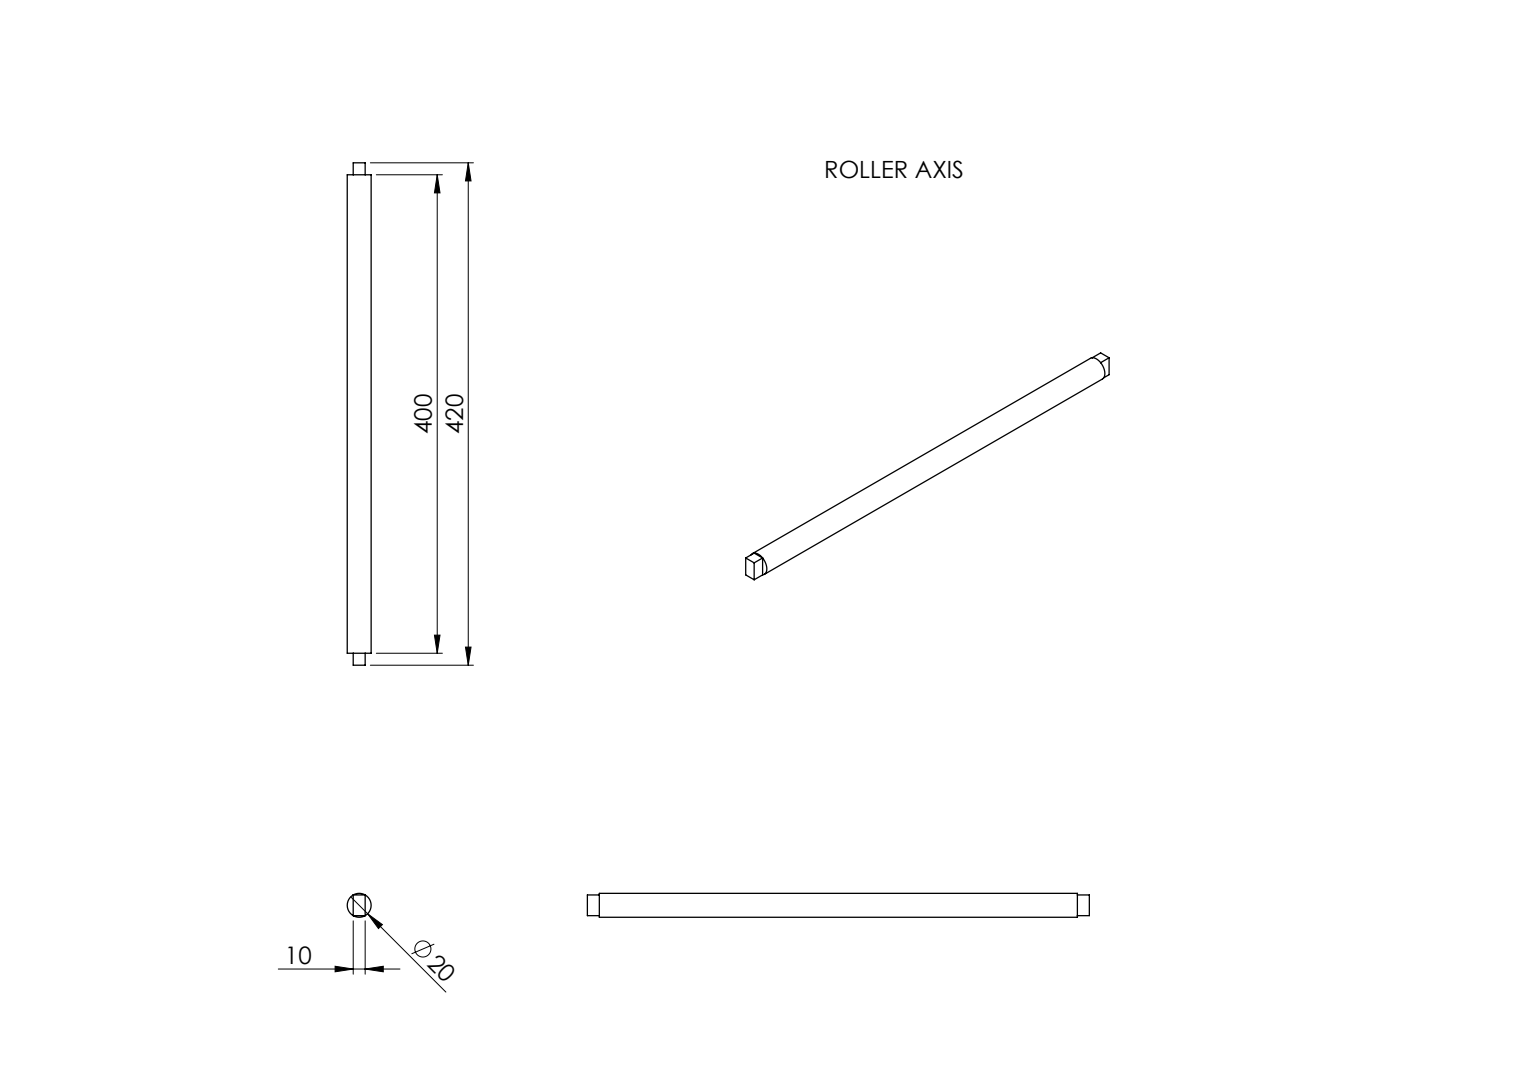
ISO-10303-21;
HEADER;
FILE_DESCRIPTION (('STEP AP214'),
    '1' );
FILE_NAME ('roller axis.step',
    '2026-10-24T13:33:06',
    ( '' ),
    ( '' ),
    'SwSTEP 2.0',
    'SolidWorks 2026',
    '' );
FILE_SCHEMA (( 'AUTOMOTIVE_DESIGN' ));
ENDSEC;

DATA;
#26=COLOUR_RGB ( '',0.8941176470588234615, 0.8941176470588234615, 0.8941176470588234615 ) ;
#48=PLANE ( 'NONE',  #10641 ) ;
#72=( NAMED_UNIT ( * ) SI_UNIT ( $, .STERADIAN. ) SOLID_ANGLE_UNIT ( ) );
#74=EDGE_CURVE ( 'NONE', #2665, #8392, #9526, .T. ) ;
#100=VECTOR ( 'NONE', #4876, 1000.000000000000000 ) ;
#101=ORIENTED_EDGE ( 'NONE', *, *, #7387, .T. ) ;
#140=VERTEX_POINT ( 'NONE', #5318 ) ;
#149=AXIS2_PLACEMENT_3D ( 'NONE', #12993, #2990, #1889 ) ;
#346=AXIS2_PLACEMENT_3D ( 'NONE', #5589, #5997, #454 ) ;
#386=VECTOR ( 'NONE', #10609, 1000.000000000000000 ) ;
#408=ORIENTED_EDGE ( 'NONE', *, *, #12527, .T. ) ;
#454=DIRECTION ( 'NONE',  ( 1.000000000000000000, 0.000000000000000000, 0.000000000000000000 ) ) ;
#467=CARTESIAN_POINT ( 'NONE',  ( 4.999999999999999112, 8.660254037844390851, 210.0000000000000000 ) ) ;
#483=PLANE ( 'NONE',  #11041 ) ;
#485=VECTOR ( 'NONE', #5913, 1000.000000000000000 ) ;
#488=CARTESIAN_POINT ( 'NONE',  ( 4.999999999999997335, -8.660254037844389075, -200.0000000000000000 ) ) ;
#527=LINE ( 'NONE', #11178, #7784 ) ;
#538=SURFACE_STYLE_FILL_AREA ( #13829 ) ;
#570=ORIENTED_EDGE ( 'NONE', *, *, #8444, .F. ) ;
#585=ORIENTED_EDGE ( 'NONE', *, *, #10780, .T. ) ;
#586=VECTOR ( 'NONE', #11904, 1000.000000000000000 ) ;
#593=AXIS2_PLACEMENT_3D ( 'NONE', #467, #9356, #3452 ) ;
#615=( NAMED_UNIT ( * ) PLANE_ANGLE_UNIT ( ) SI_UNIT ( $, .RADIAN. ) );
#620=AXIS2_PLACEMENT_3D ( 'NONE', #2454, #1137, #8922 ) ;
#723=CIRCLE ( 'NONE', #11163, 10.00000000000000000 ) ;
#735=AXIS2_PLACEMENT_3D ( 'NONE', #2825, #8104, #11669 ) ;
#737=ORIENTED_EDGE ( 'NONE', *, *, #74, .T. ) ;
#754=DIRECTION ( 'NONE',  ( -0.000000000000000000, 0.000000000000000000, 1.000000000000000000 ) ) ;
#759=( LENGTH_UNIT ( ) NAMED_UNIT ( * ) SI_UNIT ( .MILLI., .METRE. ) );
#778=CARTESIAN_POINT ( 'NONE',  ( -5.000000000000000888, 8.660254037844390851, 210.0000000000000000 ) ) ;
#796=UNCERTAINTY_MEASURE_WITH_UNIT (LENGTH_MEASURE( 1.000000000000000082E-05 ), #759, 'distance_accuracy_value', 'NONE');
#818=CARTESIAN_POINT ( 'NONE',  ( -5.000000000000000888, -8.660254037844389075, -210.0000000000000000 ) ) ;
#824=CIRCLE ( 'NONE', #346, 10.00000000000000000 ) ;
#844=VECTOR ( 'NONE', #1170, 1000.000000000000000 ) ;
#866=CARTESIAN_POINT ( 'NONE',  ( -5.000000000000000888, -8.660254037844389075, -210.0000000000000000 ) ) ;
#879=CARTESIAN_POINT ( 'NONE',  ( 0.000000000000000000, 0.000000000000000000, 200.0000000000000000 ) ) ;
#882=CARTESIAN_POINT ( 'NONE',  ( -5.000000000000000888, 8.660254037844390851, 210.0000000000000000 ) ) ;
#955=ORIENTED_EDGE ( 'NONE', *, *, #10952, .T. ) ;
#1008=VERTEX_POINT ( 'NONE', #12093 ) ;
#1060=DIRECTION ( 'NONE',  ( 0.000000000000000000, -1.000000000000000000, 0.000000000000000000 ) ) ;
#1069=FACE_OUTER_BOUND ( 'NONE', #2025, .T. ) ;
#1116=DIRECTION ( 'NONE',  ( 0.000000000000000000, 1.000000000000000000, 0.000000000000000000 ) ) ;
#1128=DIRECTION ( 'NONE',  ( 0.000000000000000000, 0.000000000000000000, 1.000000000000000000 ) ) ;
#1137=DIRECTION ( 'NONE',  ( 0.000000000000000000, -1.000000000000000000, 0.000000000000000000 ) ) ;
#1170=DIRECTION ( 'NONE',  ( -0.000000000000000000, 1.000000000000000000, 0.000000000000000000 ) ) ;
#1201=VECTOR ( 'NONE', #13083, 1000.000000000000000 ) ;
#1312=VERTEX_POINT ( 'NONE', #2925 ) ;
#1320=LINE ( 'NONE', #11483, #13363 ) ;
#1338=VERTEX_POINT ( 'NONE', #3943 ) ;
#1355=APPLICATION_CONTEXT ( 'automotive_design' ) ;
#1365=VERTEX_POINT ( 'NONE', #8283 ) ;
#1435=CIRCLE ( 'NONE', #4922, 10.00000000000000000 ) ;
#1438=PRODUCT_DEFINITION_FORMATION_WITH_SPECIFIED_SOURCE ( 'ANY', '', #7946, .NOT_KNOWN. ) ;
#1444=CARTESIAN_POINT ( 'NONE',  ( 4.999999999999999112, 8.660254037844390851, 210.0000000000000000 ) ) ;
#1532=DIRECTION ( 'NONE',  ( -0.000000000000000000, -0.000000000000000000, -1.000000000000000000 ) ) ;
#1556=DIRECTION ( 'NONE',  ( 1.000000000000000000, 0.000000000000000000, -0.000000000000000000 ) ) ;
#1581=DIRECTION ( 'NONE',  ( -0.000000000000000000, 1.000000000000000000, -0.000000000000000000 ) ) ;
#1593=SHAPE_DEFINITION_REPRESENTATION ( #4610, #5332 ) ;
#1667=MECHANICAL_DESIGN_GEOMETRIC_PRESENTATION_REPRESENTATION('',(#8148),#9795);
#1682=VERTEX_POINT ( 'NONE', #1444 ) ;
#1748=DIRECTION ( 'NONE',  ( 1.000000000000000000, 0.000000000000000000, 0.000000000000000000 ) ) ;
#1752=LINE ( 'NONE', #10626, #3426 ) ;
#1770=VERTEX_POINT ( 'NONE', #1807 ) ;
#1807=CARTESIAN_POINT ( 'NONE',  ( -5.000000000000000888, 8.660254037844387298, -200.0000000000000000 ) ) ;
#1836=CIRCLE ( 'NONE', #13404, 10.00000000000000000 ) ;
#1863=ORIENTED_EDGE ( 'NONE', *, *, #9958, .T. ) ;
#1865=( NAMED_UNIT ( * ) SI_UNIT ( $, .STERADIAN. ) SOLID_ANGLE_UNIT ( ) );
#1889=DIRECTION ( 'NONE',  ( 1.000000000000000000, 0.000000000000000000, 0.000000000000000000 ) ) ;
#1898=EDGE_LOOP ( 'NONE', ( #8131, #4401, #5922 ) ) ;
#1942=ORIENTED_EDGE ( 'NONE', *, *, #7387, .F. ) ;
#1976=CARTESIAN_POINT ( 'NONE',  ( 0.000000000000000000, 0.000000000000000000, 200.0000000000000000 ) ) ;
#1980=ADVANCED_FACE ( 'NONE', ( #3271 ), #7602, .F. ) ;
#1998=CIRCLE ( 'NONE', #11968, 10.00000000000000000 ) ;
#2019=VERTEX_POINT ( 'NONE', #818 ) ;
#2025=EDGE_LOOP ( 'NONE', ( #10502, #12176, #5270, #9510 ) ) ;
#2029=ORIENTED_EDGE ( 'NONE', *, *, #10050, .T. ) ;
#2044=ORIENTED_EDGE ( 'NONE', *, *, #7068, .F. ) ;
#2140=EDGE_CURVE ( 'NONE', #1008, #8392, #4629, .T. ) ;
#2185=ORIENTED_EDGE ( 'NONE', *, *, #8419, .F. ) ;
#2258=ORIENTED_EDGE ( 'NONE', *, *, #2140, .F. ) ;
#2282=DIRECTION ( 'NONE',  ( 0.000000000000000000, 0.000000000000000000, 1.000000000000000000 ) ) ;
#2284=( NAMED_UNIT ( * ) PLANE_ANGLE_UNIT ( ) SI_UNIT ( $, .RADIAN. ) );
#2297=DIRECTION ( 'NONE',  ( 0.000000000000000000, -0.000000000000000000, 1.000000000000000000 ) ) ;
#2298=VERTEX_POINT ( 'NONE', #12150 ) ;
#2347=DIRECTION ( 'NONE',  ( 1.000000000000000000, 0.000000000000000000, 0.000000000000000000 ) ) ;
#2421=CARTESIAN_POINT ( 'NONE',  ( 0.000000000000000000, 0.000000000000000000, 200.0000000000000000 ) ) ;
#2454=CARTESIAN_POINT ( 'NONE',  ( -5.000000000000000888, 8.660254037844390851, 210.0000000000000000 ) ) ;
#2462=AXIS2_PLACEMENT_3D ( 'NONE', #4826, #4337, #8760 ) ;
#2465=VECTOR ( 'NONE', #6841, 1000.000000000000000 ) ;
#2486=DIRECTION ( 'NONE',  ( 0.000000000000000000, 0.000000000000000000, 1.000000000000000000 ) ) ;
#2497=ORIENTED_EDGE ( 'NONE', *, *, #12527, .F. ) ;
#2518=CARTESIAN_POINT ( 'NONE',  ( -10.00000000000000000, 0.000000000000000000, 200.0000000000000000 ) ) ;
#2546=EDGE_LOOP ( 'NONE', ( #3601, #2044, #10898, #13528 ) ) ;
#2549=AXIS2_PLACEMENT_3D ( 'NONE', #11659, #5286, #9704 ) ;
#2633=ORIENTED_EDGE ( 'NONE', *, *, #4794, .T. ) ;
#2665=VERTEX_POINT ( 'NONE', #488 ) ;
#2692=FACE_OUTER_BOUND ( 'NONE', #10415, .T. ) ;
#2780=ORIENTED_EDGE ( 'NONE', *, *, #12164, .F. ) ;
#2790=DIRECTION ( 'NONE',  ( 0.000000000000000000, 0.000000000000000000, 1.000000000000000000 ) ) ;
#2819=ORIENTED_EDGE ( 'NONE', *, *, #2883, .F. ) ;
#2825=CARTESIAN_POINT ( 'NONE',  ( 0.000000000000000000, 0.000000000000000000, -200.0000000000000000 ) ) ;
#2875=ORIENTED_EDGE ( 'NONE', *, *, #7194, .T. ) ;
#2882=PLANE ( 'NONE',  #4905 ) ;
#2883=EDGE_CURVE ( 'NONE', #1770, #10068, #9446, .T. ) ;
#2904=LINE ( 'NONE', #11533, #13046 ) ;
#2925=CARTESIAN_POINT ( 'NONE',  ( -5.000000000000000888, 8.660254037844390851, 200.0000000000000000 ) ) ;
#2954=CIRCLE ( 'NONE', #11066, 10.00000000000000000 ) ;
#2971=( LENGTH_UNIT ( ) NAMED_UNIT ( * ) SI_UNIT ( .MILLI., .METRE. ) );
#2990=DIRECTION ( 'NONE',  ( 0.000000000000000000, 0.000000000000000000, 1.000000000000000000 ) ) ;
#3023=FACE_OUTER_BOUND ( 'NONE', #12665, .T. ) ;
#3065=EDGE_CURVE ( 'NONE', #3461, #2019, #13474, .T. ) ;
#3081=EDGE_LOOP ( 'NONE', ( #7439, #4815, #4294 ) ) ;
#3094=ORIENTED_EDGE ( 'NONE', *, *, #10824, .F. ) ;
#3115=FACE_OUTER_BOUND ( 'NONE', #10481, .T. ) ;
#3195=ORIENTED_EDGE ( 'NONE', *, *, #12164, .T. ) ;
#3240=CARTESIAN_POINT ( 'NONE',  ( 4.999999999999999112, -8.660254037844389075, 210.0000000000000000 ) ) ;
#3271=FACE_OUTER_BOUND ( 'NONE', #6543, .T. ) ;
#3294=LINE ( 'NONE', #5533, #13814 ) ;
#3356=FACE_OUTER_BOUND ( 'NONE', #6908, .T. ) ;
#3374=VECTOR ( 'NONE', #6254, 1000.000000000000000 ) ;
#3395=PLANE ( 'NONE',  #8036 ) ;
#3422=PLANE ( 'NONE',  #7552 ) ;
#3424=CARTESIAN_POINT ( 'NONE',  ( 0.000000000000000000, 0.000000000000000000, -200.0000000000000000 ) ) ;
#3426=VECTOR ( 'NONE', #5119, 1000.000000000000000 ) ;
#3448=DIRECTION ( 'NONE',  ( 1.000000000000000000, 0.000000000000000000, -0.000000000000000000 ) ) ;
#3452=DIRECTION ( 'NONE',  ( 0.000000000000000000, 0.000000000000000000, 1.000000000000000000 ) ) ;
#3461=VERTEX_POINT ( 'NONE', #8073 ) ;
#3494=AXIS2_PLACEMENT_3D ( 'NONE', #9933, #1128, #7019 ) ;
#3529=ORIENTED_EDGE ( 'NONE', *, *, #13666, .F. ) ;
#3531=CARTESIAN_POINT ( 'NONE',  ( 4.999999999999999112, 0.000000000000000000, -200.0000000000000000 ) ) ;
#3532=DIRECTION ( 'NONE',  ( 0.000000000000000000, 0.000000000000000000, 1.000000000000000000 ) ) ;
#3601=ORIENTED_EDGE ( 'NONE', *, *, #5962, .F. ) ;
#3633=CARTESIAN_POINT ( 'NONE',  ( 0.000000000000000000, 0.000000000000000000, -200.0000000000000000 ) ) ;
#3659=EDGE_CURVE ( 'NONE', #7893, #2298, #11709, .T. ) ;
#3712=CARTESIAN_POINT ( 'NONE',  ( -5.000000000000000888, -8.660254037844389075, 210.0000000000000000 ) ) ;
#3779=VECTOR ( 'NONE', #5752, 1000.000000000000000 ) ;
#3892=MECHANICAL_DESIGN_GEOMETRIC_PRESENTATION_REPRESENTATION('',(#13607),#11305);
#3943=CARTESIAN_POINT ( 'NONE',  ( 4.999999999999999112, 8.660254037844390851, -210.0000000000000000 ) ) ;
#3978=SURFACE_SIDE_STYLE ('',( #538 ) ) ;
#3981=CARTESIAN_POINT ( 'NONE',  ( 0.000000000000000000, 0.000000000000000000, 200.0000000000000000 ) ) ;
#4012=ADVANCED_FACE ( 'NONE', ( #1069 ), #48, .F. ) ;
#4013=AXIS2_PLACEMENT_3D ( 'NONE', #882, #7437, #4253 ) ;
#4046=ADVANCED_FACE ( 'NONE', ( #13337 ), #4367, .F. ) ;
#4119=VECTOR ( 'NONE', #10380, 1000.000000000000000 ) ;
#4121=FACE_OUTER_BOUND ( 'NONE', #14146, .T. ) ;
#4227=ORIENTED_EDGE ( 'NONE', *, *, #6491, .T. ) ;
#4250=LINE ( 'NONE', #8665, #1201 ) ;
#4253=DIRECTION ( 'NONE',  ( -0.000000000000000000, 0.000000000000000000, -1.000000000000000000 ) ) ;
#4294=ORIENTED_EDGE ( 'NONE', *, *, #3659, .T. ) ;
#4306=FACE_OUTER_BOUND ( 'NONE', #3081, .T. ) ;
#4337=DIRECTION ( 'NONE',  ( 0.000000000000000000, 0.000000000000000000, 1.000000000000000000 ) ) ;
#4338=VECTOR ( 'NONE', #1748, 1000.000000000000000 ) ;
#4352=DIRECTION ( 'NONE',  ( 0.000000000000000000, -1.000000000000000000, 0.000000000000000000 ) ) ;
#4358=CARTESIAN_POINT ( 'NONE',  ( 4.999999999999999112, 8.660254037844390851, -210.0000000000000000 ) ) ;
#4367=PLANE ( 'NONE',  #11108 ) ;
#4373=ORIENTED_EDGE ( 'NONE', *, *, #12655, .T. ) ;
#4376=ORIENTED_EDGE ( 'NONE', *, *, #6491, .F. ) ;
#4401=ORIENTED_EDGE ( 'NONE', *, *, #10040, .F. ) ;
#4436=DIRECTION ( 'NONE',  ( 1.000000000000000000, 0.000000000000000000, 0.000000000000000000 ) ) ;
#4462=LINE ( 'NONE', #3240, #8398 ) ;
#4506=CARTESIAN_POINT ( 'NONE',  ( -5.000000000000000888, -8.660254037844389075, 210.0000000000000000 ) ) ;
#4546=CARTESIAN_POINT ( 'NONE',  ( -5.000000000000000888, -8.660254037844389075, 210.0000000000000000 ) ) ;
#4573=FACE_OUTER_BOUND ( 'NONE', #11043, .T. ) ;
#4604=LINE ( 'NONE', #4749, #11744 ) ;
#4610=PRODUCT_DEFINITION_SHAPE ( 'NONE', 'NONE',  #5767 ) ;
#4617=DIRECTION ( 'NONE',  ( 0.000000000000000000, 0.000000000000000000, 1.000000000000000000 ) ) ;
#4629=CIRCLE ( 'NONE', #2549, 10.00000000000000000 ) ;
#4653=ORIENTED_EDGE ( 'NONE', *, *, #12321, .F. ) ;
#4660=DIRECTION ( 'NONE',  ( 0.000000000000000000, 0.000000000000000000, 1.000000000000000000 ) ) ;
#4694=CARTESIAN_POINT ( 'NONE',  ( 0.000000000000000000, 0.000000000000000000, -200.0000000000000000 ) ) ;
#4733=EDGE_LOOP ( 'NONE', ( #12124, #570 ) ) ;
#4749=CARTESIAN_POINT ( 'NONE',  ( -5.000000000000000888, 0.000000000000000000, 200.0000000000000000 ) ) ;
#4794=EDGE_CURVE ( 'NONE', #1770, #1008, #1836, .T. ) ;
#4800=CARTESIAN_POINT ( 'NONE',  ( -5.000000000000000888, 8.660254037844390851, 210.0000000000000000 ) ) ;
#4806=VECTOR ( 'NONE', #1581, 1000.000000000000000 ) ;
#4810=PRODUCT_CONTEXT ( 'NONE', #1355, 'mechanical' ) ;
#4815=ORIENTED_EDGE ( 'NONE', *, *, #5573, .T. ) ;
#4826=CARTESIAN_POINT ( 'NONE',  ( 0.000000000000000000, 0.000000000000000000, -200.0000000000000000 ) ) ;
#4876=DIRECTION ( 'NONE',  ( -0.000000000000000000, -0.000000000000000000, -1.000000000000000000 ) ) ;
#4900=VECTOR ( 'NONE', #5260, 1000.000000000000000 ) ;
#4905=AXIS2_PLACEMENT_3D ( 'NONE', #7292, #5346, #6210 ) ;
#4922=AXIS2_PLACEMENT_3D ( 'NONE', #3981, #6009, #5082 ) ;
#4941=ORIENTED_EDGE ( 'NONE', *, *, #8419, .T. ) ;
#4947=ORIENTED_EDGE ( 'NONE', *, *, #10119, .T. ) ;
#4948=CARTESIAN_POINT ( 'NONE',  ( 0.000000000000000000, 0.000000000000000000, -200.0000000000000000 ) ) ;
#5049=DIRECTION ( 'NONE',  ( 0.000000000000000000, 0.000000000000000000, 1.000000000000000000 ) ) ;
#5077=DIRECTION ( 'NONE',  ( 1.000000000000000000, 0.000000000000000000, 0.000000000000000000 ) ) ;
#5082=DIRECTION ( 'NONE',  ( 1.000000000000000000, 0.000000000000000000, 0.000000000000000000 ) ) ;
#5119=DIRECTION ( 'NONE',  ( -0.000000000000000000, -0.000000000000000000, -1.000000000000000000 ) ) ;
#5183=VERTEX_POINT ( 'NONE', #12368 ) ;
#5184=ORIENTED_EDGE ( 'NONE', *, *, #2140, .T. ) ;
#5260=DIRECTION ( 'NONE',  ( 0.000000000000000000, -1.000000000000000000, 0.000000000000000000 ) ) ;
#5270=ORIENTED_EDGE ( 'NONE', *, *, #13523, .F. ) ;
#5286=DIRECTION ( 'NONE',  ( 0.000000000000000000, 0.000000000000000000, 1.000000000000000000 ) ) ;
#5318=CARTESIAN_POINT ( 'NONE',  ( -4.999999999999997335, -8.660254037844389075, 200.0000000000000000 ) ) ;
#5331=CARTESIAN_POINT ( 'NONE',  ( -5.000000000000000888, 0.000000000000000000, -200.0000000000000000 ) ) ;
#5332=SHAPE_REPRESENTATION ( 'roller axis', ( #14039 ), #5930 ) ;
#5339=ADVANCED_FACE ( 'NONE', ( #13877 ), #7428, .F. ) ;
#5346=DIRECTION ( 'NONE',  ( 0.000000000000000000, 0.000000000000000000, 1.000000000000000000 ) ) ;
#5390=UNCERTAINTY_MEASURE_WITH_UNIT (LENGTH_MEASURE( 1.000000000000000082E-05 ), #2971, 'distance_accuracy_value', 'NONE');
#5426=PLANE ( 'NONE',  #2462 ) ;
#5460=CARTESIAN_POINT ( 'NONE',  ( 0.000000000000000000, 0.000000000000000000, 200.0000000000000000 ) ) ;
#5505=PLANE ( 'NONE',  #3494 ) ;
#5510=EDGE_CURVE ( 'NONE', #8392, #1770, #8879, .T. ) ;
#5533=CARTESIAN_POINT ( 'NONE',  ( -10.00000000000000000, 0.000000000000000000, 200.0000000000000000 ) ) ;
#5573=EDGE_CURVE ( 'NONE', #5764, #7893, #13370, .T. ) ;
#5583=PLANE ( 'NONE',  #620 ) ;
#5588=DIRECTION ( 'NONE',  ( 0.000000000000000000, 0.000000000000000000, 1.000000000000000000 ) ) ;
#5589=CARTESIAN_POINT ( 'NONE',  ( 0.000000000000000000, 0.000000000000000000, 200.0000000000000000 ) ) ;
#5618=AXIS2_PLACEMENT_3D ( 'NONE', #4694, #3532, #12445 ) ;
#5663=CLOSED_SHELL ( 'NONE', ( #7647, #13693, #11161, #10643, #13584, #9247, #4046, #7128, #7882, #6141, #6242, #12978, #8492, #1980, #5339, #6413, #8533, #10409, #4012, #11415 ) ) ;
#5691=EDGE_LOOP ( 'NONE', ( #7337, #955 ) ) ;
#5752=DIRECTION ( 'NONE',  ( -1.000000000000000000, 0.000000000000000000, 0.000000000000000000 ) ) ;
#5764=VERTEX_POINT ( 'NONE', #13998 ) ;
#5767=PRODUCT_DEFINITION ( 'UNKNOWN', '', #1438, #9711 ) ;
#5884=CARTESIAN_POINT ( 'NONE',  ( -5.000000000000000888, -8.660254037844389075, 210.0000000000000000 ) ) ;
#5913=DIRECTION ( 'NONE',  ( -0.000000000000000000, -0.000000000000000000, -1.000000000000000000 ) ) ;
#5922=ORIENTED_EDGE ( 'NONE', *, *, #12648, .F. ) ;
#5930=( GEOMETRIC_REPRESENTATION_CONTEXT ( 3 ) GLOBAL_UNCERTAINTY_ASSIGNED_CONTEXT ( ( #796 ) ) GLOBAL_UNIT_ASSIGNED_CONTEXT ( ( #759, #615, #1865 ) ) REPRESENTATION_CONTEXT ( 'NONE', 'WORKASPACE' ) );
#5952=LINE ( 'NONE', #4800, #100 ) ;
#5962=EDGE_CURVE ( 'NONE', #1312, #7893, #527, .T. ) ;
#5967=EDGE_CURVE ( 'NONE', #140, #2298, #824, .T. ) ;
#5997=DIRECTION ( 'NONE',  ( 0.000000000000000000, 0.000000000000000000, 1.000000000000000000 ) ) ;
#6009=DIRECTION ( 'NONE',  ( 0.000000000000000000, 0.000000000000000000, 1.000000000000000000 ) ) ;
#6049=VECTOR ( 'NONE', #13178, 1000.000000000000000 ) ;
#6141=ADVANCED_FACE ( 'NONE', ( #3356 ), #12054, .T. ) ;
#6190=AXIS2_PLACEMENT_3D ( 'NONE', #1976, #8509, #7558 ) ;
#6195=CARTESIAN_POINT ( 'NONE',  ( 4.999999999999999112, 0.000000000000000000, 200.0000000000000000 ) ) ;
#6210=DIRECTION ( 'NONE',  ( 1.000000000000000000, 0.000000000000000000, -0.000000000000000000 ) ) ;
#6242=ADVANCED_FACE ( 'NONE', ( #4573 ), #3422, .F. ) ;
#6254=DIRECTION ( 'NONE',  ( -1.000000000000000000, 0.000000000000000000, 0.000000000000000000 ) ) ;
#6272=CIRCLE ( 'NONE', #12760, 10.00000000000000000 ) ;
#6344=UNCERTAINTY_MEASURE_WITH_UNIT (LENGTH_MEASURE( 1.000000000000000082E-05 ), #6635, 'distance_accuracy_value', 'NONE');
#6345=PLANE ( 'NONE',  #6190 ) ;
#6405=ORIENTED_EDGE ( 'NONE', *, *, #7442, .T. ) ;
#6413=ADVANCED_FACE ( 'NONE', ( #12544 ), #8105, .F. ) ;
#6439=CIRCLE ( 'NONE', #149, 10.00000000000000000 ) ;
#6491=EDGE_CURVE ( 'NONE', #140, #1312, #4604, .T. ) ;
#6495=PLANE ( 'NONE',  #4013 ) ;
#6543=EDGE_LOOP ( 'NONE', ( #12547, #7520, #9847, #101 ) ) ;
#6599=CARTESIAN_POINT ( 'NONE',  ( -5.000000000000000888, 8.660254037844390851, 210.0000000000000000 ) ) ;
#6635=( LENGTH_UNIT ( ) NAMED_UNIT ( * ) SI_UNIT ( .MILLI., .METRE. ) );
#6693=EDGE_LOOP ( 'NONE', ( #7933, #737, #4941, #14118 ) ) ;
#6745=DIRECTION ( 'NONE',  ( -1.000000000000000000, 0.000000000000000000, 0.000000000000000000 ) ) ;
#6796=FACE_OUTER_BOUND ( 'NONE', #6693, .T. ) ;
#6814=DIRECTION ( 'NONE',  ( -0.000000000000000000, -0.000000000000000000, -1.000000000000000000 ) ) ;
#6827=DIRECTION ( 'NONE',  ( 1.000000000000000000, 0.000000000000000000, -0.000000000000000000 ) ) ;
#6841=DIRECTION ( 'NONE',  ( -0.000000000000000000, -0.000000000000000000, -1.000000000000000000 ) ) ;
#6866=ORIENTED_EDGE ( 'NONE', *, *, #9534, .F. ) ;
#6870=FACE_OUTER_BOUND ( 'NONE', #10927, .T. ) ;
#6878=FACE_OUTER_BOUND ( 'NONE', #2546, .T. ) ;
#6908=EDGE_LOOP ( 'NONE', ( #2780, #6866, #7688, #11826, #408, #5184, #7968, #8995 ) ) ;
#6909=ORIENTED_EDGE ( 'NONE', *, *, #11653, .F. ) ;
#6915=DIRECTION ( 'NONE',  ( -0.000000000000000000, 1.000000000000000000, 0.000000000000000000 ) ) ;
#6966=LINE ( 'NONE', #8118, #4806 ) ;
#7019=DIRECTION ( 'NONE',  ( 1.000000000000000000, 0.000000000000000000, -0.000000000000000000 ) ) ;
#7056=CARTESIAN_POINT ( 'NONE',  ( 10.00000000000000000, 1.224646799147353256E-15, 200.0000000000000000 ) ) ;
#7068=EDGE_CURVE ( 'NONE', #1365, #1312, #5952, .T. ) ;
#7103=CARTESIAN_POINT ( 'NONE',  ( 0.000000000000000000, -8.660254037844389075, 200.0000000000000000 ) ) ;
#7118=AXIS2_PLACEMENT_3D ( 'NONE', #5460, #11054, #6827 ) ;
#7128=ADVANCED_FACE ( 'NONE', ( #2692 ), #483, .F. ) ;
#7194=EDGE_CURVE ( 'NONE', #10963, #1338, #9867, .T. ) ;
#7205=DIRECTION ( 'NONE',  ( 1.000000000000000000, 0.000000000000000000, 0.000000000000000000 ) ) ;
#7292=CARTESIAN_POINT ( 'NONE',  ( 0.000000000000000000, 0.000000000000000000, -200.0000000000000000 ) ) ;
#7337=ORIENTED_EDGE ( 'NONE', *, *, #5967, .T. ) ;
#7351=AXIS2_PLACEMENT_3D ( 'NONE', #778, #13061, #12116 ) ;
#7367=CARTESIAN_POINT ( 'NONE',  ( 0.000000000000000000, 0.000000000000000000, -200.0000000000000000 ) ) ;
#7378=DIRECTION ( 'NONE',  ( -1.000000000000000000, 0.000000000000000000, 0.000000000000000000 ) ) ;
#7379=SHAPE_REPRESENTATION_RELATIONSHIP ( 'NONE' , 'NONE' ,  #5332, #13210 ) ;
#7387=EDGE_CURVE ( 'NONE', #1338, #3461, #8847, .T. ) ;
#7428=PLANE ( 'NONE',  #8539 ) ;
#7437=DIRECTION ( 'NONE',  ( 1.000000000000000000, 0.000000000000000000, -0.000000000000000000 ) ) ;
#7439=ORIENTED_EDGE ( 'NONE', *, *, #9534, .T. ) ;
#7442=EDGE_CURVE ( 'NONE', #1365, #13895, #13331, .T. ) ;
#7520=ORIENTED_EDGE ( 'NONE', *, *, #2883, .T. ) ;
#7529=CARTESIAN_POINT ( 'NONE',  ( -5.000000000000000888, 8.660254037844390851, 210.0000000000000000 ) ) ;
#7552=AXIS2_PLACEMENT_3D ( 'NONE', #7683, #12183, #4436 ) ;
#7558=DIRECTION ( 'NONE',  ( 1.000000000000000000, 0.000000000000000000, -0.000000000000000000 ) ) ;
#7602=PLANE ( 'NONE',  #9266 ) ;
#7647=ADVANCED_FACE ( 'NONE', ( #3115 ), #8393, .T. ) ;
#7675=EDGE_LOOP ( 'NONE', ( #2819, #8630 ) ) ;
#7683=CARTESIAN_POINT ( 'NONE',  ( 0.000000000000000000, 0.000000000000000000, -210.0000000000000000 ) ) ;
#7688=ORIENTED_EDGE ( 'NONE', *, *, #5967, .F. ) ;
#7784=VECTOR ( 'NONE', #1556, 1000.000000000000000 ) ;
#7826=DIRECTION ( 'NONE',  ( 1.000000000000000000, 0.000000000000000000, -0.000000000000000000 ) ) ;
#7882=ADVANCED_FACE ( 'NONE', ( #10324 ), #5426, .F. ) ;
#7893=VERTEX_POINT ( 'NONE', #13182 ) ;
#7933=ORIENTED_EDGE ( 'NONE', *, *, #10050, .F. ) ;
#7946=PRODUCT ( 'roller axis', 'roller axis', '', ( #4810 ) ) ;
#7960=ORIENTED_EDGE ( 'NONE', *, *, #7194, .F. ) ;
#7968=ORIENTED_EDGE ( 'NONE', *, *, #8444, .T. ) ;
#7969=DIRECTION ( 'NONE',  ( 1.000000000000000000, 0.000000000000000000, 0.000000000000000000 ) ) ;
#8036=AXIS2_PLACEMENT_3D ( 'NONE', #4546, #1116, #2297 ) ;
#8073=CARTESIAN_POINT ( 'NONE',  ( -5.000000000000000888, 8.660254037844390851, -210.0000000000000000 ) ) ;
#8103=CARTESIAN_POINT ( 'NONE',  ( -5.000000000000000888, 8.660254037844390851, -210.0000000000000000 ) ) ;
#8104=DIRECTION ( 'NONE',  ( 0.000000000000000000, 0.000000000000000000, 1.000000000000000000 ) ) ;
#8105=PLANE ( 'NONE',  #593 ) ;
#8118=CARTESIAN_POINT ( 'NONE',  ( 4.999999999999999112, 8.660254037844390851, 210.0000000000000000 ) ) ;
#8131=ORIENTED_EDGE ( 'NONE', *, *, #11656, .F. ) ;
#8148=STYLED_ITEM ( 'NONE', ( #13758 ), #13210 ) ;
#8239=( NAMED_UNIT ( * ) PLANE_ANGLE_UNIT ( ) SI_UNIT ( $, .RADIAN. ) );
#8283=CARTESIAN_POINT ( 'NONE',  ( -5.000000000000000888, 8.660254037844390851, 210.0000000000000000 ) ) ;
#8357=VERTEX_POINT ( 'NONE', #13925 ) ;
#8372=PLANE ( 'NONE',  #9803 ) ;
#8392=VERTEX_POINT ( 'NONE', #10607 ) ;
#8393=CYLINDRICAL_SURFACE ( 'NONE', #8956, 10.00000000000000000 ) ;
#8398=VECTOR ( 'NONE', #8885, 1000.000000000000000 ) ;
#8419=EDGE_CURVE ( 'NONE', #8392, #2019, #13856, .T. ) ;
#8426=LINE ( 'NONE', #12854, #9901 ) ;
#8444=EDGE_CURVE ( 'NONE', #8392, #2665, #6439, .T. ) ;
#8492=ADVANCED_FACE ( 'NONE', ( #9733 ), #8639, .F. ) ;
#8509=DIRECTION ( 'NONE',  ( 0.000000000000000000, 0.000000000000000000, 1.000000000000000000 ) ) ;
#8533=ADVANCED_FACE ( 'NONE', ( #6878 ), #5583, .F. ) ;
#8539=AXIS2_PLACEMENT_3D ( 'NONE', #11785, #12644, #5049 ) ;
#8557=ORIENTED_EDGE ( 'NONE', *, *, #12273, .T. ) ;
#8621=CIRCLE ( 'NONE', #5618, 10.00000000000000000 ) ;
#8630=ORIENTED_EDGE ( 'NONE', *, *, #10119, .F. ) ;
#8639=PLANE ( 'NONE',  #7351 ) ;
#8648=EDGE_LOOP ( 'NONE', ( #11208, #9016, #2029, #2875 ) ) ;
#8665=CARTESIAN_POINT ( 'NONE',  ( -5.000000000000000888, 8.660254037844390851, 210.0000000000000000 ) ) ;
#8677=ORIENTED_EDGE ( 'NONE', *, *, #9958, .F. ) ;
#8723=DIRECTION ( 'NONE',  ( -0.000000000000000000, -0.000000000000000000, -1.000000000000000000 ) ) ;
#8757=DIRECTION ( 'NONE',  ( 1.000000000000000000, 0.000000000000000000, 0.000000000000000000 ) ) ;
#8760=DIRECTION ( 'NONE',  ( 1.000000000000000000, 0.000000000000000000, -0.000000000000000000 ) ) ;
#8775=CARTESIAN_POINT ( 'NONE',  ( -5.000000000000000888, 8.660254037844390851, -210.0000000000000000 ) ) ;
#8813=DIRECTION ( 'NONE',  ( 1.000000000000000000, 0.000000000000000000, 0.000000000000000000 ) ) ;
#8847=LINE ( 'NONE', #8775, #9644 ) ;
#8879=LINE ( 'NONE', #5331, #844 ) ;
#8885=DIRECTION ( 'NONE',  ( -0.000000000000000000, -0.000000000000000000, -1.000000000000000000 ) ) ;
#8922=DIRECTION ( 'NONE',  ( 0.000000000000000000, -0.000000000000000000, -1.000000000000000000 ) ) ;
#8956=AXIS2_PLACEMENT_3D ( 'NONE', #11809, #14048, #7378 ) ;
#8995=ORIENTED_EDGE ( 'NONE', *, *, #12648, .T. ) ;
#9004=VERTEX_POINT ( 'NONE', #2518 ) ;
#9016=ORIENTED_EDGE ( 'NONE', *, *, #11656, .T. ) ;
#9029=ORIENTED_EDGE ( 'NONE', *, *, #10040, .T. ) ;
#9031=LINE ( 'NONE', #3531, #6049 ) ;
#9033=CARTESIAN_POINT ( 'NONE',  ( 4.999999999999993783, 8.660254037844390851, -200.0000000000000000 ) ) ;
#9110=CARTESIAN_POINT ( 'NONE',  ( 4.999999999999999112, -8.660254037844389075, 210.0000000000000000 ) ) ;
#9247=ADVANCED_FACE ( 'NONE', ( #13968 ), #2882, .F. ) ;
#9251=ORIENTED_EDGE ( 'NONE', *, *, #5510, .F. ) ;
#9266=AXIS2_PLACEMENT_3D ( 'NONE', #7529, #4352, #11967 ) ;
#9267=ORIENTED_EDGE ( 'NONE', *, *, #5510, .T. ) ;
#9356=DIRECTION ( 'NONE',  ( -1.000000000000000000, 0.000000000000000000, 0.000000000000000000 ) ) ;
#9367=DIRECTION ( 'NONE',  ( 1.000000000000000000, 0.000000000000000000, -0.000000000000000000 ) ) ;
#9392=ORIENTED_EDGE ( 'NONE', *, *, #5573, .F. ) ;
#9418=DIRECTION ( 'NONE',  ( 0.000000000000000000, 0.000000000000000000, 1.000000000000000000 ) ) ;
#9446=LINE ( 'NONE', #11687, #386 ) ;
#9461=DIRECTION ( 'NONE',  ( 1.000000000000000000, 0.000000000000000000, 0.000000000000000000 ) ) ;
#9510=ORIENTED_EDGE ( 'NONE', *, *, #10824, .T. ) ;
#9526=LINE ( 'NONE', #11771, #3374 ) ;
#9534=EDGE_CURVE ( 'NONE', #2298, #5764, #723, .T. ) ;
#9644=VECTOR ( 'NONE', #12388, 1000.000000000000000 ) ;
#9681=FACE_OUTER_BOUND ( 'NONE', #5691, .T. ) ;
#9704=DIRECTION ( 'NONE',  ( 1.000000000000000000, 0.000000000000000000, 0.000000000000000000 ) ) ;
#9710=CARTESIAN_POINT ( 'NONE',  ( 0.000000000000000000, 0.000000000000000000, 210.0000000000000000 ) ) ;
#9711=PRODUCT_DEFINITION_CONTEXT ( 'detailed design', #13047, 'design' ) ;
#9733=FACE_OUTER_BOUND ( 'NONE', #10616, .T. ) ;
#9779=PLANE ( 'NONE',  #13226 ) ;
#9795=( GEOMETRIC_REPRESENTATION_CONTEXT ( 3 ) GLOBAL_UNCERTAINTY_ASSIGNED_CONTEXT ( ( #5390 ) ) GLOBAL_UNIT_ASSIGNED_CONTEXT ( ( #2971, #8239, #12674 ) ) REPRESENTATION_CONTEXT ( 'NONE', 'WORKASPACE' ) );
#9796=ORIENTED_EDGE ( 'NONE', *, *, #11653, .T. ) ;
#9803=AXIS2_PLACEMENT_3D ( 'NONE', #879, #12807, #3448 ) ;
#9847=ORIENTED_EDGE ( 'NONE', *, *, #12447, .T. ) ;
#9867=LINE ( 'NONE', #4358, #586 ) ;
#9884=ORIENTED_EDGE ( 'NONE', *, *, #7442, .F. ) ;
#9886=EDGE_LOOP ( 'NONE', ( #12408, #3529, #12840, #12139 ) ) ;
#9901=VECTOR ( 'NONE', #13008, 1000.000000000000000 ) ;
#9933=CARTESIAN_POINT ( 'NONE',  ( 0.000000000000000000, 0.000000000000000000, 200.0000000000000000 ) ) ;
#9948=DIRECTION ( 'NONE',  ( 0.000000000000000000, 1.000000000000000000, 0.000000000000000000 ) ) ;
#9958=EDGE_CURVE ( 'NONE', #1312, #9004, #1435, .T. ) ;
#10040=EDGE_CURVE ( 'NONE', #8357, #10068, #13024, .T. ) ;
#10050=EDGE_CURVE ( 'NONE', #2665, #10963, #13519, .T. ) ;
#10068=VERTEX_POINT ( 'NONE', #9033 ) ;
#10080=DIRECTION ( 'NONE',  ( 0.000000000000000000, -0.000000000000000000, 1.000000000000000000 ) ) ;
#10119=EDGE_CURVE ( 'NONE', #10068, #1770, #8621, .T. ) ;
#10123=CARTESIAN_POINT ( 'NONE',  ( 0.000000000000000000, 0.000000000000000000, 200.0000000000000000 ) ) ;
#10324=FACE_OUTER_BOUND ( 'NONE', #4733, .T. ) ;
#10371=ORIENTED_EDGE ( 'NONE', *, *, #3065, .F. ) ;
#10380=DIRECTION ( 'NONE',  ( -0.000000000000000000, -0.000000000000000000, -1.000000000000000000 ) ) ;
#10394=LINE ( 'NONE', #7056, #2465 ) ;
#10409=ADVANCED_FACE ( 'NONE', ( #3023 ), #6495, .F. ) ;
#10415=EDGE_LOOP ( 'NONE', ( #9251, #2258, #11399 ) ) ;
#10438=VECTOR ( 'NONE', #11383, 1000.000000000000000 ) ;
#10481=EDGE_LOOP ( 'NONE', ( #9392, #3195, #9029, #4947, #2633, #2497, #8677, #6909 ) ) ;
#10502=ORIENTED_EDGE ( 'NONE', *, *, #10952, .F. ) ;
#10508=CARTESIAN_POINT ( 'NONE',  ( 0.000000000000000000, 0.000000000000000000, 0.000000000000000000 ) ) ;
#10567=DIRECTION ( 'NONE',  ( 0.000000000000000000, 0.000000000000000000, 1.000000000000000000 ) ) ;
#10607=CARTESIAN_POINT ( 'NONE',  ( -5.000000000000000888, -8.660254037844389075, -200.0000000000000284 ) ) ;
#10609=DIRECTION ( 'NONE',  ( 1.000000000000000000, 0.000000000000000000, -0.000000000000000000 ) ) ;
#10616=EDGE_LOOP ( 'NONE', ( #2185, #9267, #8557, #13119 ) ) ;
#10626=CARTESIAN_POINT ( 'NONE',  ( 4.999999999999999112, 8.660254037844390851, 210.0000000000000000 ) ) ;
#10641=AXIS2_PLACEMENT_3D ( 'NONE', #4506, #9948, #10080 ) ;
#10643=ADVANCED_FACE ( 'NONE', ( #13882 ), #8372, .T. ) ;
#10655=FILL_AREA_STYLE_COLOUR ( '', #26 ) ;
#10670=EDGE_CURVE ( 'NONE', #5183, #2298, #4462, .T. ) ;
#10693=ORIENTED_EDGE ( 'NONE', *, *, #12000, .T. ) ;
#10780=EDGE_CURVE ( 'NONE', #1682, #1365, #4250, .T. ) ;
#10824=EDGE_CURVE ( 'NONE', #13895, #140, #2904, .T. ) ;
#10898=ORIENTED_EDGE ( 'NONE', *, *, #10780, .F. ) ;
#10927=EDGE_LOOP ( 'NONE', ( #9796, #11629 ) ) ;
#10941=DIRECTION ( 'NONE',  ( 1.000000000000000000, 0.000000000000000000, 0.000000000000000000 ) ) ;
#10952=EDGE_CURVE ( 'NONE', #2298, #140, #12361, .T. ) ;
#10963=VERTEX_POINT ( 'NONE', #14269 ) ;
#11041=AXIS2_PLACEMENT_3D ( 'NONE', #4948, #12769, #9367 ) ;
#11043=EDGE_LOOP ( 'NONE', ( #7960, #4653, #10371, #1942 ) ) ;
#11054=DIRECTION ( 'NONE',  ( 0.000000000000000000, 0.000000000000000000, 1.000000000000000000 ) ) ;
#11066=AXIS2_PLACEMENT_3D ( 'NONE', #3633, #4660, #7969 ) ;
#11108=AXIS2_PLACEMENT_3D ( 'NONE', #3424, #5588, #7826 ) ;
#11161=ADVANCED_FACE ( 'NONE', ( #6870 ), #5505, .T. ) ;
#11163=AXIS2_PLACEMENT_3D ( 'NONE', #12721, #2790, #7205 ) ;
#11178=CARTESIAN_POINT ( 'NONE',  ( 0.000000000000000000, 8.660254037844390851, 200.0000000000000000 ) ) ;
#11208=ORIENTED_EDGE ( 'NONE', *, *, #12447, .F. ) ;
#11287=AXIS2_PLACEMENT_3D ( 'NONE', #13566, #2486, #2347 ) ;
#11305=( GEOMETRIC_REPRESENTATION_CONTEXT ( 3 ) GLOBAL_UNCERTAINTY_ASSIGNED_CONTEXT ( ( #6344 ) ) GLOBAL_UNIT_ASSIGNED_CONTEXT ( ( #6635, #2284, #72 ) ) REPRESENTATION_CONTEXT ( 'NONE', 'WORKASPACE' ) );
#11321=ORIENTED_EDGE ( 'NONE', *, *, #13523, .T. ) ;
#11383=DIRECTION ( 'NONE',  ( 0.000000000000000000, -1.000000000000000000, 0.000000000000000000 ) ) ;
#11399=ORIENTED_EDGE ( 'NONE', *, *, #4794, .F. ) ;
#11415=ADVANCED_FACE ( 'NONE', ( #4121 ), #9779, .T. ) ;
#11483=CARTESIAN_POINT ( 'NONE',  ( -5.000000000000000888, 8.660254037844390851, 210.0000000000000000 ) ) ;
#11496=VECTOR ( 'NONE', #1060, 1000.000000000000000 ) ;
#11502=AXIS2_PLACEMENT_3D ( 'NONE', #13275, #6814, #6745 ) ;
#11533=CARTESIAN_POINT ( 'NONE',  ( -5.000000000000000888, -8.660254037844389075, 210.0000000000000000 ) ) ;
#11629=ORIENTED_EDGE ( 'NONE', *, *, #5962, .T. ) ;
#11653=EDGE_CURVE ( 'NONE', #7893, #1312, #6272, .T. ) ;
#11656=EDGE_CURVE ( 'NONE', #10068, #2665, #9031, .T. ) ;
#11659=CARTESIAN_POINT ( 'NONE',  ( 0.000000000000000000, 0.000000000000000000, -200.0000000000000000 ) ) ;
#11669=DIRECTION ( 'NONE',  ( 1.000000000000000000, 0.000000000000000000, 0.000000000000000000 ) ) ;
#11687=CARTESIAN_POINT ( 'NONE',  ( 0.000000000000000000, 8.660254037844390851, -200.0000000000000000 ) ) ;
#11709=LINE ( 'NONE', #6195, #4900 ) ;
#11744=VECTOR ( 'NONE', #6915, 1000.000000000000000 ) ;
#11771=CARTESIAN_POINT ( 'NONE',  ( 0.000000000000000000, -8.660254037844389075, -200.0000000000000000 ) ) ;
#11780=CARTESIAN_POINT ( 'NONE',  ( -5.000000000000000888, -8.660254037844389075, 210.0000000000000000 ) ) ;
#11785=CARTESIAN_POINT ( 'NONE',  ( 4.999999999999999112, 8.660254037844390851, 210.0000000000000000 ) ) ;
#11809=CARTESIAN_POINT ( 'NONE',  ( 0.000000000000000000, 0.000000000000000000, 200.0000000000000000 ) ) ;
#11826=ORIENTED_EDGE ( 'NONE', *, *, #12000, .F. ) ;
#11904=DIRECTION ( 'NONE',  ( -0.000000000000000000, 1.000000000000000000, -0.000000000000000000 ) ) ;
#11967=DIRECTION ( 'NONE',  ( 0.000000000000000000, -0.000000000000000000, -1.000000000000000000 ) ) ;
#11968=AXIS2_PLACEMENT_3D ( 'NONE', #2421, #2282, #8813 ) ;
#12000=EDGE_CURVE ( 'NONE', #9004, #140, #1998, .T. ) ;
#12054=CYLINDRICAL_SURFACE ( 'NONE', #11502, 10.00000000000000000 ) ;
#12069=PLANE ( 'NONE',  #7118 ) ;
#12093=CARTESIAN_POINT ( 'NONE',  ( -10.00000000000000000, 0.000000000000000000, -200.0000000000000000 ) ) ;
#12116=DIRECTION ( 'NONE',  ( -0.000000000000000000, 0.000000000000000000, -1.000000000000000000 ) ) ;
#12124=ORIENTED_EDGE ( 'NONE', *, *, #74, .F. ) ;
#12139=ORIENTED_EDGE ( 'NONE', *, *, #10670, .T. ) ;
#12150=CARTESIAN_POINT ( 'NONE',  ( 4.999999999999999112, -8.660254037844389075, 200.0000000000000000 ) ) ;
#12164=EDGE_CURVE ( 'NONE', #5764, #8357, #10394, .T. ) ;
#12176=ORIENTED_EDGE ( 'NONE', *, *, #10670, .F. ) ;
#12183=DIRECTION ( 'NONE',  ( -0.000000000000000000, 0.000000000000000000, 1.000000000000000000 ) ) ;
#12273=EDGE_CURVE ( 'NONE', #1770, #3461, #1320, .T. ) ;
#12321=EDGE_CURVE ( 'NONE', #2019, #10963, #13508, .T. ) ;
#12361=LINE ( 'NONE', #7103, #3779 ) ;
#12368=CARTESIAN_POINT ( 'NONE',  ( 4.999999999999999112, -8.660254037844389075, 210.0000000000000000 ) ) ;
#12388=DIRECTION ( 'NONE',  ( -1.000000000000000000, -0.000000000000000000, -0.000000000000000000 ) ) ;
#12408=ORIENTED_EDGE ( 'NONE', *, *, #3659, .F. ) ;
#12445=DIRECTION ( 'NONE',  ( 1.000000000000000000, 0.000000000000000000, 0.000000000000000000 ) ) ;
#12447=EDGE_CURVE ( 'NONE', #10068, #1338, #8426, .T. ) ;
#12468=VECTOR ( 'NONE', #9461, 1000.000000000000000 ) ;
#12527=EDGE_CURVE ( 'NONE', #9004, #1008, #3294, .T. ) ;
#12544=FACE_OUTER_BOUND ( 'NONE', #9886, .T. ) ;
#12547=ORIENTED_EDGE ( 'NONE', *, *, #12273, .F. ) ;
#12644=DIRECTION ( 'NONE',  ( -1.000000000000000000, 0.000000000000000000, 0.000000000000000000 ) ) ;
#12648=EDGE_CURVE ( 'NONE', #2665, #8357, #2954, .T. ) ;
#12655=EDGE_CURVE ( 'NONE', #5183, #1682, #6966, .T. ) ;
#12665=EDGE_LOOP ( 'NONE', ( #4376, #3094, #9884, #14149 ) ) ;
#12674=( NAMED_UNIT ( * ) SI_UNIT ( $, .STERADIAN. ) SOLID_ANGLE_UNIT ( ) );
#12721=CARTESIAN_POINT ( 'NONE',  ( 0.000000000000000000, 0.000000000000000000, 200.0000000000000000 ) ) ;
#12760=AXIS2_PLACEMENT_3D ( 'NONE', #10123, #4617, #8757 ) ;
#12769=DIRECTION ( 'NONE',  ( 0.000000000000000000, 0.000000000000000000, 1.000000000000000000 ) ) ;
#12807=DIRECTION ( 'NONE',  ( 0.000000000000000000, 0.000000000000000000, 1.000000000000000000 ) ) ;
#12840=ORIENTED_EDGE ( 'NONE', *, *, #12655, .F. ) ;
#12854=CARTESIAN_POINT ( 'NONE',  ( 4.999999999999999112, 8.660254037844390851, 210.0000000000000000 ) ) ;
#12954=DIRECTION ( 'NONE',  ( 1.000000000000000000, 0.000000000000000000, 0.000000000000000000 ) ) ;
#12978=ADVANCED_FACE ( 'NONE', ( #6796 ), #3395, .F. ) ;
#12993=CARTESIAN_POINT ( 'NONE',  ( 0.000000000000000000, 0.000000000000000000, -200.0000000000000000 ) ) ;
#13008=DIRECTION ( 'NONE',  ( -0.000000000000000000, -0.000000000000000000, -1.000000000000000000 ) ) ;
#13024=CIRCLE ( 'NONE', #735, 10.00000000000000000 ) ;
#13046=VECTOR ( 'NONE', #13915, 1000.000000000000000 ) ;
#13047=APPLICATION_CONTEXT ( 'automotive_design' ) ;
#13061=DIRECTION ( 'NONE',  ( 1.000000000000000000, 0.000000000000000000, -0.000000000000000000 ) ) ;
#13083=DIRECTION ( 'NONE',  ( -1.000000000000000000, -0.000000000000000000, -0.000000000000000000 ) ) ;
#13119=ORIENTED_EDGE ( 'NONE', *, *, #3065, .T. ) ;
#13178=DIRECTION ( 'NONE',  ( 0.000000000000000000, -1.000000000000000000, 0.000000000000000000 ) ) ;
#13182=CARTESIAN_POINT ( 'NONE',  ( 4.999999999999999112, 8.660254037844390851, 200.0000000000000000 ) ) ;
#13210=ADVANCED_BREP_SHAPE_REPRESENTATION ( '', ( #13385, #14039 ), #5930 ) ;
#13226=AXIS2_PLACEMENT_3D ( 'NONE', #9710, #754, #10941 ) ;
#13275=CARTESIAN_POINT ( 'NONE',  ( 0.000000000000000000, 0.000000000000000000, 200.0000000000000000 ) ) ;
#13331=LINE ( 'NONE', #6599, #11496 ) ;
#13337=FACE_OUTER_BOUND ( 'NONE', #7675, .T. ) ;
#13363=VECTOR ( 'NONE', #1532, 1000.000000000000000 ) ;
#13370=CIRCLE ( 'NONE', #11287, 10.00000000000000000 ) ;
#13385=MANIFOLD_SOLID_BREP ( 'Boss-Extrude2', #5663 ) ;
#13404=AXIS2_PLACEMENT_3D ( 'NONE', #7367, #10567, #12954 ) ;
#13474=LINE ( 'NONE', #8103, #10438 ) ;
#13508=LINE ( 'NONE', #866, #4338 ) ;
#13519=LINE ( 'NONE', #9110, #485 ) ;
#13523=EDGE_CURVE ( 'NONE', #13895, #5183, #14157, .T. ) ;
#13528=ORIENTED_EDGE ( 'NONE', *, *, #13666, .T. ) ;
#13566=CARTESIAN_POINT ( 'NONE',  ( 0.000000000000000000, 0.000000000000000000, 200.0000000000000000 ) ) ;
#13584=ADVANCED_FACE ( 'NONE', ( #9681 ), #6345, .T. ) ;
#13607=STYLED_ITEM('',(#14403),#13385);
#13666=EDGE_CURVE ( 'NONE', #1682, #7893, #1752, .T. ) ;
#13693=ADVANCED_FACE ( 'NONE', ( #4306 ), #12069, .T. ) ;
#13758=PRESENTATION_STYLE_ASSIGNMENT (( #14050 ) ) ;
#13814=VECTOR ( 'NONE', #8723, 1000.000000000000000 ) ;
#13829=FILL_AREA_STYLE ('',( #10655 ) ) ;
#13856=LINE ( 'NONE', #3712, #4119 ) ;
#13877=FACE_OUTER_BOUND ( 'NONE', #8648, .T. ) ;
#13882=FACE_OUTER_BOUND ( 'NONE', #14168, .T. ) ;
#13895=VERTEX_POINT ( 'NONE', #5884 ) ;
#13915=DIRECTION ( 'NONE',  ( -0.000000000000000000, -0.000000000000000000, -1.000000000000000000 ) ) ;
#13925=CARTESIAN_POINT ( 'NONE',  ( 10.00000000000000000, 1.224646799147353256E-15, -200.0000000000000000 ) ) ;
#13968=FACE_OUTER_BOUND ( 'NONE', #1898, .T. ) ;
#13998=CARTESIAN_POINT ( 'NONE',  ( 10.00000000000000000, 1.224646799147353256E-15, 200.0000000000000000 ) ) ;
#14039=AXIS2_PLACEMENT_3D ( 'NONE', #10508, #9418, #5077 ) ;
#14048=DIRECTION ( 'NONE',  ( -0.000000000000000000, -0.000000000000000000, -1.000000000000000000 ) ) ;
#14050=SURFACE_STYLE_USAGE ( .BOTH. , #3978 ) ;
#14118=ORIENTED_EDGE ( 'NONE', *, *, #12321, .T. ) ;
#14146=EDGE_LOOP ( 'NONE', ( #4373, #585, #6405, #11321 ) ) ;
#14149=ORIENTED_EDGE ( 'NONE', *, *, #7068, .T. ) ;
#14157=LINE ( 'NONE', #11780, #12468 ) ;
#14168=EDGE_LOOP ( 'NONE', ( #1863, #10693, #4227 ) ) ;
#14269=CARTESIAN_POINT ( 'NONE',  ( 4.999999999999999112, -8.660254037844389075, -210.0000000000000000 ) ) ;
#14397=COLOUR_RGB('Sky Blue',0.24,0.69,0.87);
#14398=FILL_AREA_STYLE_COLOUR('',#14397);
#14399=FILL_AREA_STYLE('',(#14398));
#14400=SURFACE_STYLE_FILL_AREA(#14399);
#14401=SURFACE_SIDE_STYLE('',(#14400));
#14402=SURFACE_STYLE_USAGE(.BOTH.,#14401);
#14403=PRESENTATION_STYLE_ASSIGNMENT((#14402));
ENDSEC;
END-ISO-10303-21;
